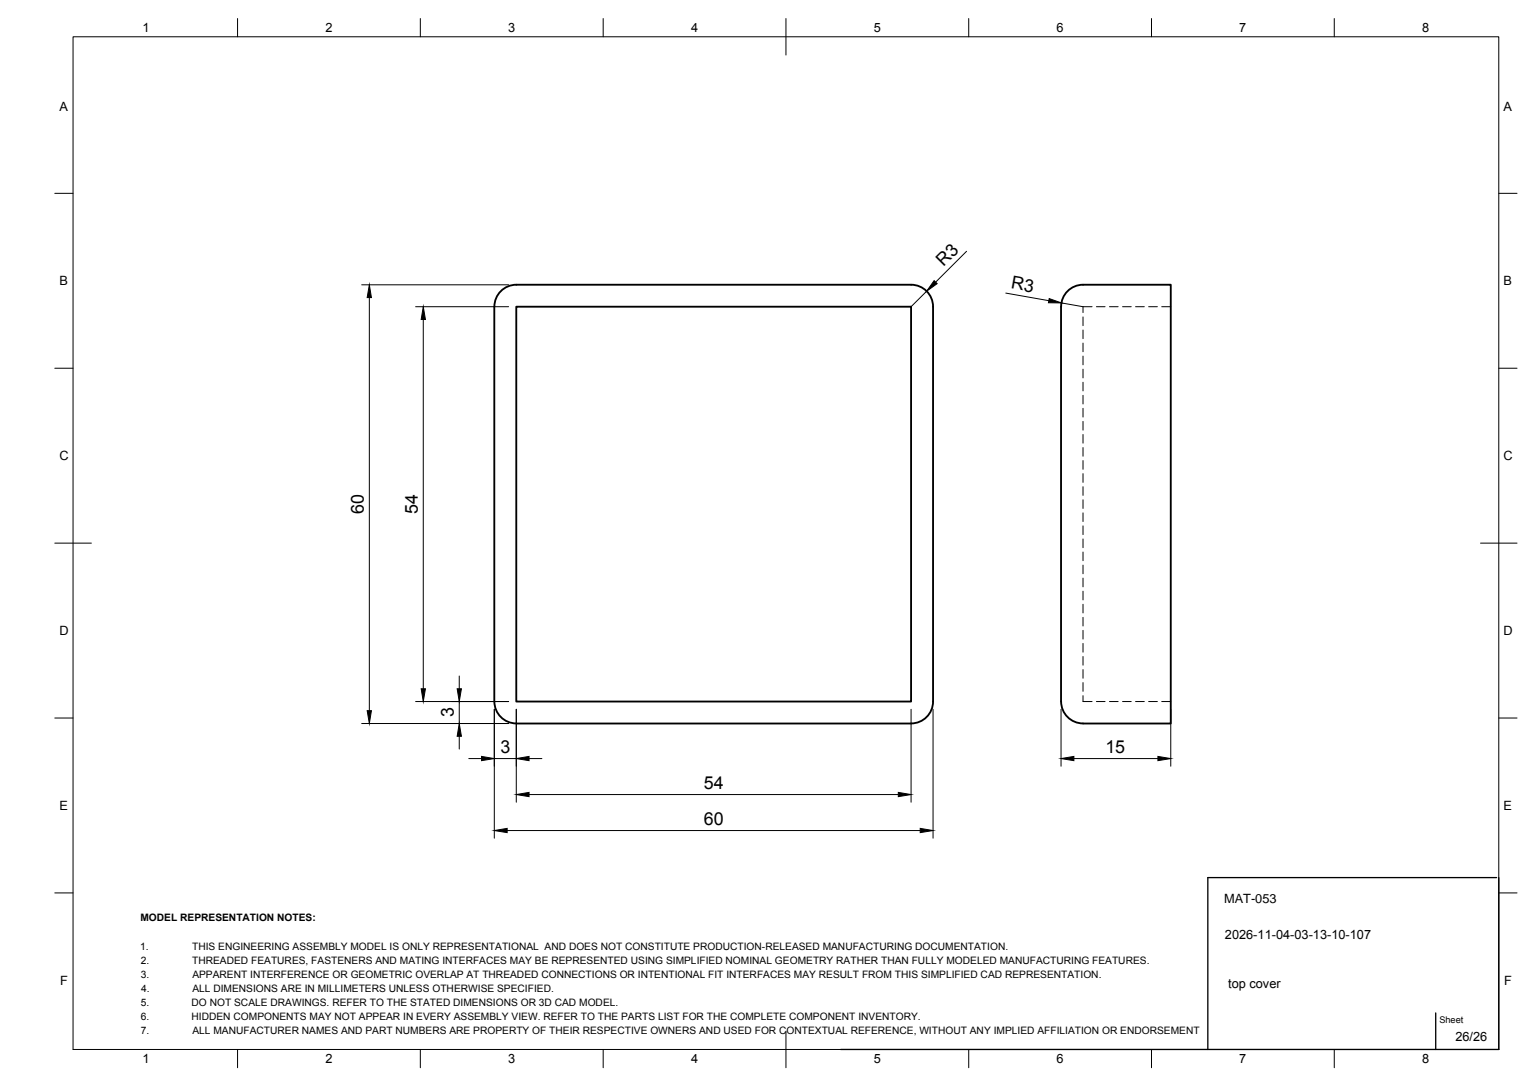
ISO-10303-21;
HEADER;
FILE_DESCRIPTION (('STEP AP214'),
    '1' );
FILE_NAME ('top cover.step',
    '2026-10-10T03:43:58',
    ( '' ),
    ( '' ),
    'SwSTEP 2.0',
    'SolidWorks 2026',
    '' );
FILE_SCHEMA (( 'AUTOMOTIVE_DESIGN' ));
ENDSEC;

DATA;
#205=DIRECTION ( 'NONE',  ( 0.000000000000000000, 0.000000000000000000, -1.000000000000000000 ) ) ;
#232=CARTESIAN_POINT ( 'NONE',  ( -30.00000000000000355, 26.99999999999999289, 12.00000000000000000 ) ) ;
#298=DIRECTION ( 'NONE',  ( 0.000000000000000000, 1.000000000000000000, 0.000000000000000000 ) ) ;
#580=CARTESIAN_POINT ( 'NONE',  ( 0.000000000000000000, 0.000000000000000000, 0.000000000000000000 ) ) ;
#658=DIRECTION ( 'NONE',  ( 0.000000000000000000, 1.000000000000000000, 0.000000000000000000 ) ) ;
#710=ORIENTED_EDGE ( 'NONE', *, *, #12281, .T. ) ;
#818=VECTOR ( 'NONE', #14052, 1000.000000000000000 ) ;
#1029=CARTESIAN_POINT ( 'NONE',  ( 26.99999999999999645, -27.00000000000000355, 12.00000000000000000 ) ) ;
#1414=ORIENTED_EDGE ( 'NONE', *, *, #50736, .T. ) ;
#1463=DIRECTION ( 'NONE',  ( 0.000000000000000000, -1.000000000000000000, 0.000000000000000000 ) ) ;
#1569=CARTESIAN_POINT ( 'NONE',  ( 26.99999999999999645, 0.000000000000000000, 15.00000000000000000 ) ) ;
#1686=CIRCLE ( 'NONE', #47705, 2.999999999999999112 ) ;
#1835=CARTESIAN_POINT ( 'NONE',  ( -27.00000000000000355, -27.00000000000000355, 15.00000000000000000 ) ) ;
#1860=LINE ( 'NONE', #18024, #9010 ) ;
#1950=ORIENTED_EDGE ( 'NONE', *, *, #16118, .F. ) ;
#2102=ORIENTED_EDGE ( 'NONE', *, *, #62336, .T. ) ;
#2271=FACE_OUTER_BOUND ( 'NONE', #44764, .T. ) ;
#2303=EDGE_CURVE ( 'NONE', #6058, #28877, #22222, .T. ) ;
#2927=ORIENTED_EDGE ( 'NONE', *, *, #30408, .T. ) ;
#3081=AXIS2_PLACEMENT_3D ( 'NONE', #1029, #66114, #17904 ) ;
#3101=EDGE_LOOP ( 'NONE', ( #24985, #13574, #25623 ) ) ;
#3252=DIRECTION ( 'NONE',  ( 0.000000000000000000, -1.000000000000000000, 0.000000000000000000 ) ) ;
#3314=EDGE_CURVE ( 'NONE', #69327, #44889, #32443, .T. ) ;
#3324=DIRECTION ( 'NONE',  ( -0.000000000000000000, -0.000000000000000000, -1.000000000000000000 ) ) ;
#3439=ADVANCED_FACE ( 'NONE', ( #7097 ), #12728, .T. ) ;
#3520=CARTESIAN_POINT ( 'NONE',  ( 26.99999999999999645, 0.000000000000000000, -0.000000000000000000 ) ) ;
#3667=CARTESIAN_POINT ( 'NONE',  ( -27.00000000000000355, 26.99999999999999645, 0.000000000000000000 ) ) ;
#3801=DIRECTION ( 'NONE',  ( -1.000000000000000000, -1.156482317317871725E-15, 0.000000000000000000 ) ) ;
#3891=ORIENTED_EDGE ( 'NONE', *, *, #46841, .F. ) ;
#4008=ORIENTED_EDGE ( 'NONE', *, *, #30408, .F. ) ;
#4241=EDGE_CURVE ( 'NONE', #32499, #62713, #15839, .T. ) ;
#4403=ORIENTED_EDGE ( 'NONE', *, *, #17309, .T. ) ;
#4446=DIRECTION ( 'NONE',  ( 0.000000000000000000, 0.000000000000000000, -1.000000000000000000 ) ) ;
#4489=LINE ( 'NONE', #19627, #58799 ) ;
#4810=DIRECTION ( 'NONE',  ( 0.000000000000000000, 0.000000000000000000, 1.000000000000000000 ) ) ;
#4904=EDGE_CURVE ( 'NONE', #26503, #8633, #55459, .T. ) ;
#5040=CARTESIAN_POINT ( 'NONE',  ( 29.99999999999999645, -27.00000000000000355, 15.00000000000000000 ) ) ;
#5156=ORIENTED_EDGE ( 'NONE', *, *, #23205, .T. ) ;
#5210=PLANE ( 'NONE',  #52619 ) ;
#5318=DIRECTION ( 'NONE',  ( 0.000000000000000000, 0.000000000000000000, -1.000000000000000000 ) ) ;
#5366=AXIS2_PLACEMENT_3D ( 'NONE', #65979, #17774, #7580 ) ;
#5409=ORIENTED_EDGE ( 'NONE', *, *, #63357, .T. ) ;
#5648=CARTESIAN_POINT ( 'NONE',  ( -27.00000000000000355, 26.99999999999999289, 0.000000000000000000 ) ) ;
#5733=VECTOR ( 'NONE', #47729, 1000.000000000000000 ) ;
#5803=ORIENTED_EDGE ( 'NONE', *, *, #46794, .F. ) ;
#5843=DIRECTION ( 'NONE',  ( -1.000000000000000000, 0.000000000000000000, -0.000000000000000000 ) ) ;
#5940=CARTESIAN_POINT ( 'NONE',  ( 26.99999999999999289, -30.00000000000000355, 0.000000000000000000 ) ) ;
#5961=DIRECTION ( 'NONE',  ( 0.000000000000000000, 0.000000000000000000, -1.000000000000000000 ) ) ;
#6058=VERTEX_POINT ( 'NONE', #3667 ) ;
#6102=ORIENTED_EDGE ( 'NONE', *, *, #58756, .F. ) ;
#6143=DIRECTION ( 'NONE',  ( 0.000000000000000000, 0.000000000000000000, -1.000000000000000000 ) ) ;
#6198=FACE_OUTER_BOUND ( 'NONE', #21474, .T. ) ;
#6225=VERTEX_POINT ( 'NONE', #41647 ) ;
#6428=VECTOR ( 'NONE', #48833, 1000.000000000000000 ) ;
#6478=ORIENTED_EDGE ( 'NONE', *, *, #62336, .F. ) ;
#6480=ORIENTED_EDGE ( 'NONE', *, *, #50724, .F. ) ;
#6516=EDGE_CURVE ( 'NONE', #6225, #40175, #1686, .T. ) ;
#6716=FACE_OUTER_BOUND ( 'NONE', #43158, .T. ) ;
#6823=CARTESIAN_POINT ( 'NONE',  ( 0.000000000000000000, -27.00000000000000355, 15.00000000000000000 ) ) ;
#6825=DIRECTION ( 'NONE',  ( -0.000000000000000000, -0.000000000000000000, 1.000000000000000000 ) ) ;
#6889=ORIENTED_EDGE ( 'NONE', *, *, #66647, .F. ) ;
#7011=DIRECTION ( 'NONE',  ( 1.000000000000000000, 0.000000000000000000, 0.000000000000000000 ) ) ;
#7097=FACE_OUTER_BOUND ( 'NONE', #42212, .T. ) ;
#7102=VECTOR ( 'NONE', #45225, 1000.000000000000000 ) ;
#7438=ORIENTED_EDGE ( 'NONE', *, *, #22139, .T. ) ;
#7471=CIRCLE ( 'NONE', #49967, 2.999999999999999112 ) ;
#7580=DIRECTION ( 'NONE',  ( 0.000000000000000000, -0.000000000000000000, -1.000000000000000000 ) ) ;
#7623=AXIS2_PLACEMENT_3D ( 'NONE', #12347, #50333, #60872 ) ;
#7667=VERTEX_POINT ( 'NONE', #19524 ) ;
#7674=CARTESIAN_POINT ( 'NONE',  ( 26.99999999999999289, 26.99999999999999645, 12.00000000000000000 ) ) ;
#8001=LINE ( 'NONE', #29456, #37178 ) ;
#8141=CARTESIAN_POINT ( 'NONE',  ( -27.00000000000000355, -30.00000000000000355, 15.00000000000000000 ) ) ;
#8234=CYLINDRICAL_SURFACE ( 'NONE', #53074, 2.999999999999999112 ) ;
#8319=DIRECTION ( 'NONE',  ( 1.000000000000000000, 0.000000000000000000, 0.000000000000000000 ) ) ;
#8334=FACE_OUTER_BOUND ( 'NONE', #46485, .T. ) ;
#8423=ADVANCED_FACE ( 'NONE', ( #66101 ), #17538, .F. ) ;
#8496=LINE ( 'NONE', #45780, #36770 ) ;
#8633=VERTEX_POINT ( 'NONE', #11470 ) ;
#8718=AXIS2_PLACEMENT_3D ( 'NONE', #29906, #55232, #39077 ) ;
#8728=FACE_OUTER_BOUND ( 'NONE', #54277, .T. ) ;
#8810=ORIENTED_EDGE ( 'NONE', *, *, #54510, .T. ) ;
#8945=ORIENTED_EDGE ( 'NONE', *, *, #65993, .T. ) ;
#9010=VECTOR ( 'NONE', #54598, 1000.000000000000000 ) ;
#9074=PRODUCT_DEFINITION_SHAPE ( 'NONE', 'NONE',  #55565 ) ;
#9081=VERTEX_POINT ( 'NONE', #5940 ) ;
#9480=EDGE_CURVE ( 'NONE', #41324, #25791, #48125, .T. ) ;
#9811=CIRCLE ( 'NONE', #12060, 2.999999999999999112 ) ;
#9857=ADVANCED_FACE ( 'NONE', ( #21322 ), #65637, .T. ) ;
#9955=PRODUCT_DEFINITION_CONTEXT ( 'detailed design', #26937, 'design' ) ;
#10261=CARTESIAN_POINT ( 'NONE',  ( 26.99999999999999645, 26.99999999999999645, 12.00000000000000000 ) ) ;
#10445=CARTESIAN_POINT ( 'NONE',  ( 26.99999999999999645, 26.99999999999999645, 12.00000000000000000 ) ) ;
#10700=ADVANCED_FACE ( 'NONE', ( #6716 ), #19613, .T. ) ;
#10784=ADVANCED_FACE ( 'NONE', ( #8728 ), #33803, .T. ) ;
#10889=CIRCLE ( 'NONE', #3081, 2.999999999999999112 ) ;
#11030=CARTESIAN_POINT ( 'NONE',  ( 26.99999999999999645, -30.00000000000000355, 15.00000000000000000 ) ) ;
#11039=ORIENTED_EDGE ( 'NONE', *, *, #23029, .T. ) ;
#11086=ORIENTED_EDGE ( 'NONE', *, *, #66647, .T. ) ;
#11217=LINE ( 'NONE', #32684, #6428 ) ;
#11234=VECTOR ( 'NONE', #23749, 1000.000000000000000 ) ;
#11470=CARTESIAN_POINT ( 'NONE',  ( -30.00000000000000355, -27.00000000000000355, 0.000000000000000000 ) ) ;
#11537=PLANE ( 'NONE',  #37652 ) ;
#12060=AXIS2_PLACEMENT_3D ( 'NONE', #26984, #27675, #49116 ) ;
#12281=EDGE_CURVE ( 'NONE', #9081, #43408, #15395, .T. ) ;
#12347=CARTESIAN_POINT ( 'NONE',  ( -30.00000000000000355, 26.99999999999999645, 15.00000000000000000 ) ) ;
#12478=LINE ( 'NONE', #1569, #18550 ) ;
#12484=CARTESIAN_POINT ( 'NONE',  ( -30.00000000000000355, -27.00000000000000355, 12.00000000000000000 ) ) ;
#12728=CYLINDRICAL_SURFACE ( 'NONE', #65623, 2.999999999999999112 ) ;
#12815=UNCERTAINTY_MEASURE_WITH_UNIT (LENGTH_MEASURE( 1.000000000000000082E-05 ), #48462, 'distance_accuracy_value', 'NONE');
#12853=DIRECTION ( 'NONE',  ( -0.000000000000000000, -0.000000000000000000, 1.000000000000000000 ) ) ;
#12906=ADVANCED_FACE ( 'NONE', ( #19001 ), #17611, .T. ) ;
#12964=ADVANCED_FACE ( 'NONE', ( #41498 ), #31295, .T. ) ;
#13056=CARTESIAN_POINT ( 'NONE',  ( 29.99999999999999645, -30.00000000000000355, 15.00000000000000000 ) ) ;
#13156=EDGE_LOOP ( 'NONE', ( #33249, #52496, #29073, #69310 ) ) ;
#13179=VECTOR ( 'NONE', #67585, 1000.000000000000000 ) ;
#13198=CARTESIAN_POINT ( 'NONE',  ( 29.99999999999999645, 26.99999999999999289, 15.00000000000000000 ) ) ;
#13396=FACE_OUTER_BOUND ( 'NONE', #32596, .T. ) ;
#13574=ORIENTED_EDGE ( 'NONE', *, *, #33002, .T. ) ;
#13635=ADVANCED_FACE ( 'NONE', ( #13396 ), #62265, .T. ) ;
#13692=VECTOR ( 'NONE', #25426, 1000.000000000000000 ) ;
#13696=ORIENTED_EDGE ( 'NONE', *, *, #42477, .T. ) ;
#13708=ORIENTED_EDGE ( 'NONE', *, *, #25060, .F. ) ;
#13830=AXIS2_PLACEMENT_3D ( 'NONE', #48385, #55427, #44883 ) ;
#13919=CIRCLE ( 'NONE', #29629, 2.999999999999999112 ) ;
#14052=DIRECTION ( 'NONE',  ( 1.000000000000000000, 0.000000000000000000, 0.000000000000000000 ) ) ;
#14415=ORIENTED_EDGE ( 'NONE', *, *, #50724, .T. ) ;
#14417=LINE ( 'NONE', #29901, #51494 ) ;
#14459=DIRECTION ( 'NONE',  ( 0.000000000000000000, 0.000000000000000000, -1.000000000000000000 ) ) ;
#14478=CIRCLE ( 'NONE', #21293, 2.999999999999999112 ) ;
#14630=ORIENTED_EDGE ( 'NONE', *, *, #6516, .F. ) ;
#14733=VECTOR ( 'NONE', #50808, 1000.000000000000000 ) ;
#14750=DIRECTION ( 'NONE',  ( 0.000000000000000000, 0.000000000000000000, 1.000000000000000000 ) ) ;
#14758=DIRECTION ( 'NONE',  ( -1.000000000000000000, 0.000000000000000000, 0.000000000000000000 ) ) ;
#14846=CARTESIAN_POINT ( 'NONE',  ( 0.000000000000000000, 26.99999999999999645, 0.000000000000000000 ) ) ;
#14880=CARTESIAN_POINT ( 'NONE',  ( -30.00000000000000355, -30.00000000000000355, 12.00000000000000000 ) ) ;
#14925=AXIS2_PLACEMENT_3D ( 'NONE', #580, #32930, #5843 ) ;
#15172=CIRCLE ( 'NONE', #65745, 2.999999999999999112 ) ;
#15255=EDGE_LOOP ( 'NONE', ( #31860, #60299, #4403, #51256 ) ) ;
#15269=EDGE_LOOP ( 'NONE', ( #5409, #23940, #8810, #19099 ) ) ;
#15349=CARTESIAN_POINT ( 'NONE',  ( 26.99999999999999289, 26.99999999999999645, 0.000000000000000000 ) ) ;
#15395=LINE ( 'NONE', #44096, #62596 ) ;
#15581=VECTOR ( 'NONE', #57340, 1000.000000000000000 ) ;
#15839=LINE ( 'NONE', #64363, #26189 ) ;
#16028=( GEOMETRIC_REPRESENTATION_CONTEXT ( 3 ) GLOBAL_UNCERTAINTY_ASSIGNED_CONTEXT ( ( #12815 ) ) GLOBAL_UNIT_ASSIGNED_CONTEXT ( ( #48462, #43201, #37241 ) ) REPRESENTATION_CONTEXT ( 'NONE', 'WORKASPACE' ) );
#16037=DIRECTION ( 'NONE',  ( -0.000000000000000000, -1.000000000000000000, -0.000000000000000000 ) ) ;
#16118=EDGE_CURVE ( 'NONE', #6225, #52460, #57437, .T. ) ;
#16138=FILL_AREA_STYLE ('',( #37940 ) ) ;
#16158=EDGE_LOOP ( 'NONE', ( #47934, #54871, #19275, #17353 ) ) ;
#16540=DIRECTION ( 'NONE',  ( 0.000000000000000000, 0.000000000000000000, 1.000000000000000000 ) ) ;
#16832=DIRECTION ( 'NONE',  ( -1.000000000000000000, 0.000000000000000000, -0.000000000000000000 ) ) ;
#16893=CARTESIAN_POINT ( 'NONE',  ( 26.99999999999999645, -27.00000000000000355, 15.00000000000000000 ) ) ;
#17309=EDGE_CURVE ( 'NONE', #39573, #51452, #60293, .T. ) ;
#17353=ORIENTED_EDGE ( 'NONE', *, *, #38024, .F. ) ;
#17522=AXIS2_PLACEMENT_3D ( 'NONE', #10445, #68838, #3801 ) ;
#17538=PLANE ( 'NONE',  #29861 ) ;
#17561=CARTESIAN_POINT ( 'NONE',  ( -27.00000000000000355, -27.00000000000000355, 12.00000000000000000 ) ) ;
#17611=PLANE ( 'NONE',  #8718 ) ;
#17774=DIRECTION ( 'NONE',  ( 0.000000000000000000, -1.000000000000000000, 0.000000000000000000 ) ) ;
#17904=DIRECTION ( 'NONE',  ( 0.000000000000000000, 0.000000000000000000, -1.000000000000000000 ) ) ;
#18024=CARTESIAN_POINT ( 'NONE',  ( -27.00000000000000355, -30.00000000000000355, 12.00000000000000000 ) ) ;
#18121=FACE_OUTER_BOUND ( 'NONE', #15269, .T. ) ;
#18189=CARTESIAN_POINT ( 'NONE',  ( -27.00000000000000355, 0.000000000000000000, 12.00000000000000000 ) ) ;
#18295=DIRECTION ( 'NONE',  ( 0.000000000000000000, 0.000000000000000000, -1.000000000000000000 ) ) ;
#18314=DIRECTION ( 'NONE',  ( 0.000000000000000000, 0.000000000000000000, 1.000000000000000000 ) ) ;
#18380=CARTESIAN_POINT ( 'NONE',  ( -27.00000000000000355, 0.000000000000000000, 15.00000000000000000 ) ) ;
#18492=AXIS2_PLACEMENT_3D ( 'NONE', #7674, #66771, #66427 ) ;
#18550=VECTOR ( 'NONE', #66655, 1000.000000000000000 ) ;
#18804=EDGE_CURVE ( 'NONE', #8633, #64962, #45182, .T. ) ;
#19001=FACE_OUTER_BOUND ( 'NONE', #64825, .T. ) ;
#19099=ORIENTED_EDGE ( 'NONE', *, *, #46794, .T. ) ;
#19215=CYLINDRICAL_SURFACE ( 'NONE', #39889, 2.999999999999999112 ) ;
#19275=ORIENTED_EDGE ( 'NONE', *, *, #65275, .F. ) ;
#19323=VERTEX_POINT ( 'NONE', #40685 ) ;
#19413=ORIENTED_EDGE ( 'NONE', *, *, #22139, .F. ) ;
#19469=CARTESIAN_POINT ( 'NONE',  ( 26.99999999999999645, 0.000000000000000000, 12.00000000000000000 ) ) ;
#19485=CARTESIAN_POINT ( 'NONE',  ( -30.00000000000000355, -27.00000000000000355, 15.00000000000000000 ) ) ;
#19524=CARTESIAN_POINT ( 'NONE',  ( -27.00000000000000355, -30.00000000000000355, 12.00000000000000000 ) ) ;
#19613=SPHERICAL_SURFACE ( 'NONE', #23333, 3.000000000000000000 ) ;
#19627=CARTESIAN_POINT ( 'NONE',  ( -30.00000000000000355, 26.99999999999999645, 12.00000000000000000 ) ) ;
#19872=EDGE_CURVE ( 'NONE', #6225, #39573, #57397, .T. ) ;
#19906=VECTOR ( 'NONE', #12853, 1000.000000000000000 ) ;
#20346=CARTESIAN_POINT ( 'NONE',  ( -27.00000000000000355, -30.00000000000000355, 15.00000000000000000 ) ) ;
#20503=LINE ( 'NONE', #14880, #48624 ) ;
#20784=ADVANCED_FACE ( 'NONE', ( #63984 ), #43899, .T. ) ;
#20791=MANIFOLD_SOLID_BREP ( 'Shell1', #42893 ) ;
#20967=DIRECTION ( 'NONE',  ( -1.000000000000000000, 0.000000000000000000, 0.000000000000000000 ) ) ;
#21082=ORIENTED_EDGE ( 'NONE', *, *, #30023, .T. ) ;
#21293=AXIS2_PLACEMENT_3D ( 'NONE', #39648, #54767, #34030 ) ;
#21294=DIRECTION ( 'NONE',  ( -1.000000000000000000, 0.000000000000000000, 0.000000000000000000 ) ) ;
#21320=DIRECTION ( 'NONE',  ( -1.000000000000000000, -0.000000000000000000, -0.000000000000000000 ) ) ;
#21321=ADVANCED_FACE ( 'NONE', ( #59647, #38206 ), #42447, .T. ) ;
#21322=FACE_OUTER_BOUND ( 'NONE', #56192, .T. ) ;
#21333=FACE_OUTER_BOUND ( 'NONE', #52946, .T. ) ;
#21352=ADVANCED_FACE ( 'NONE', ( #6198 ), #43473, .T. ) ;
#21422=ADVANCED_FACE ( 'NONE', ( #21333 ), #26957, .T. ) ;
#21428=EDGE_CURVE ( 'NONE', #64962, #40175, #32250, .T. ) ;
#21474=EDGE_LOOP ( 'NONE', ( #13696, #62459, #1950, #30513 ) ) ;
#21793=CARTESIAN_POINT ( 'NONE',  ( -27.00000000000000355, 29.99999999999999645, 0.000000000000000000 ) ) ;
#22018=CARTESIAN_POINT ( 'NONE',  ( 26.99999999999999645, -27.00000000000000355, 15.00000000000000000 ) ) ;
#22139=EDGE_CURVE ( 'NONE', #55869, #25791, #4489, .T. ) ;
#22181=ORIENTED_EDGE ( 'NONE', *, *, #55920, .F. ) ;
#22222=LINE ( 'NONE', #28185, #62196 ) ;
#22231=DIRECTION ( 'NONE',  ( 0.000000000000000000, 0.000000000000000000, -1.000000000000000000 ) ) ;
#22375=DIRECTION ( 'NONE',  ( 0.000000000000000000, 0.000000000000000000, 1.000000000000000000 ) ) ;
#22511=CARTESIAN_POINT ( 'NONE',  ( -27.00000000000000355, -27.00000000000000355, 15.00000000000000000 ) ) ;
#22720=CARTESIAN_POINT ( 'NONE',  ( -27.00000000000000355, -27.00000000000000355, 12.00000000000000000 ) ) ;
#23029=EDGE_CURVE ( 'NONE', #7667, #26503, #45423, .T. ) ;
#23205=EDGE_CURVE ( 'NONE', #28877, #59754, #42563, .T. ) ;
#23333=AXIS2_PLACEMENT_3D ( 'NONE', #28881, #28161, #66185 ) ;
#23743=CARTESIAN_POINT ( 'NONE',  ( 29.99999999999999645, -27.00000000000000355, 0.000000000000000000 ) ) ;
#23749=DIRECTION ( 'NONE',  ( 0.000000000000000000, 0.000000000000000000, -1.000000000000000000 ) ) ;
#23940=ORIENTED_EDGE ( 'NONE', *, *, #55920, .T. ) ;
#24075=CIRCLE ( 'NONE', #18492, 2.999999999999999112 ) ;
#24302=PLANE ( 'NONE',  #33156 ) ;
#24695=ADVANCED_FACE ( 'NONE', ( #8334 ), #19215, .T. ) ;
#24734=DIRECTION ( 'NONE',  ( 0.000000000000000000, -0.000000000000000000, 1.000000000000000000 ) ) ;
#24976=EDGE_CURVE ( 'NONE', #43408, #44889, #29799, .T. ) ;
#24985=ORIENTED_EDGE ( 'NONE', *, *, #58756, .T. ) ;
#24993=STYLED_ITEM ( 'NONE', ( #58355 ), #20791 ) ;
#25060=EDGE_CURVE ( 'NONE', #51452, #42318, #12478, .T. ) ;
#25151=AXIS2_PLACEMENT_3D ( 'NONE', #31684, #69315, #60843 ) ;
#25426=DIRECTION ( 'NONE',  ( -1.000000000000000000, 0.000000000000000000, 0.000000000000000000 ) ) ;
#25582=DIRECTION ( 'NONE',  ( 0.000000000000000000, 1.000000000000000000, 0.000000000000000000 ) ) ;
#25623=ORIENTED_EDGE ( 'NONE', *, *, #50443, .F. ) ;
#25689=LINE ( 'NONE', #3520, #15581 ) ;
#25714=DIRECTION ( 'NONE',  ( 1.000000000000000000, -0.000000000000000000, 0.000000000000000000 ) ) ;
#25791=VERTEX_POINT ( 'NONE', #26067 ) ;
#25812=AXIS2_PLACEMENT_3D ( 'NONE', #28884, #50672, #29224 ) ;
#25890=PRODUCT_CONTEXT ( 'NONE', #58769, 'mechanical' ) ;
#25918=LINE ( 'NONE', #53306, #62997 ) ;
#26000=CARTESIAN_POINT ( 'NONE',  ( -27.00000000000000355, 26.99999999999999289, 12.00000000000000000 ) ) ;
#26067=CARTESIAN_POINT ( 'NONE',  ( 26.99999999999999645, 26.99999999999999645, 12.00000000000000000 ) ) ;
#26189=VECTOR ( 'NONE', #63343, 1000.000000000000000 ) ;
#26232=CYLINDRICAL_SURFACE ( 'NONE', #50132, 2.999999999999999112 ) ;
#26328=DIRECTION ( 'NONE',  ( 0.000000000000000000, 0.000000000000000000, -1.000000000000000000 ) ) ;
#26357=CARTESIAN_POINT ( 'NONE',  ( 26.99999999999999289, 29.99999999999999645, 0.000000000000000000 ) ) ;
#26389=ORIENTED_EDGE ( 'NONE', *, *, #43751, .T. ) ;
#26423=ORIENTED_EDGE ( 'NONE', *, *, #50443, .T. ) ;
#26503=VERTEX_POINT ( 'NONE', #35598 ) ;
#26528=DIRECTION ( 'NONE',  ( -1.000000000000000000, 0.000000000000000000, 0.000000000000000000 ) ) ;
#26668=DIRECTION ( 'NONE',  ( 1.000000000000000000, 0.000000000000000000, 0.000000000000000000 ) ) ;
#26860=AXIS2_PLACEMENT_3D ( 'NONE', #49201, #37972, #7011 ) ;
#26910=ADVANCED_FACE ( 'NONE', ( #61229 ), #24302, .F. ) ;
#26937=APPLICATION_CONTEXT ( 'automotive_design' ) ;
#26957=SPHERICAL_SURFACE ( 'NONE', #13830, 3.000000000000000000 ) ;
#26984=CARTESIAN_POINT ( 'NONE',  ( -27.00000000000000355, 26.99999999999999645, 12.00000000000000000 ) ) ;
#27010=ADVANCED_FACE ( 'NONE', ( #48816 ), #11537, .F. ) ;
#27026=AXIS2_PLACEMENT_3D ( 'NONE', #41140, #56624, #18295 ) ;
#27068=ORIENTED_EDGE ( 'NONE', *, *, #30420, .T. ) ;
#27182=VECTOR ( 'NONE', #54516, 1000.000000000000000 ) ;
#27248=CARTESIAN_POINT ( 'NONE',  ( -30.00000000000000355, 29.99999999999999645, 12.00000000000000000 ) ) ;
#27377=SURFACE_STYLE_FILL_AREA ( #16138 ) ;
#27456=EDGE_LOOP ( 'NONE', ( #49518, #62100, #56589, #22181 ) ) ;
#27675=DIRECTION ( 'NONE',  ( 0.000000000000000000, -0.000000000000000000, 1.000000000000000000 ) ) ;
#27696=EDGE_LOOP ( 'NONE', ( #2927, #11086, #60441, #28815 ) ) ;
#27909=PLANE ( 'NONE',  #47841 ) ;
#27999=CARTESIAN_POINT ( 'NONE',  ( -30.00000000000000355, -30.00000000000000355, 12.00000000000000000 ) ) ;
#28096=CARTESIAN_POINT ( 'NONE',  ( 26.99999999999999289, 29.99999999999999645, 15.00000000000000000 ) ) ;
#28161=DIRECTION ( 'NONE',  ( 1.000000000000000000, 0.000000000000000000, 0.000000000000000000 ) ) ;
#28185=CARTESIAN_POINT ( 'NONE',  ( -27.00000000000000355, 0.000000000000000000, -0.000000000000000000 ) ) ;
#28196=DIRECTION ( 'NONE',  ( -1.000000000000000000, 0.000000000000000000, 0.000000000000000000 ) ) ;
#28288=SHAPE_REPRESENTATION_RELATIONSHIP ( 'NONE' , 'NONE' ,  #31639, #32386 ) ;
#28319=ADVANCED_FACE ( 'NONE', ( #41781 ), #62893, .T. ) ;
#28482=EDGE_LOOP ( 'NONE', ( #6478, #66068, #6480, #57491, #36541, #8945, #38878, #60954 ) ) ;
#28660=CARTESIAN_POINT ( 'NONE',  ( 26.99999999999999645, -27.00000000000000355, 12.00000000000000000 ) ) ;
#28671=CARTESIAN_POINT ( 'NONE',  ( 26.99999999999999289, 29.99999999999999645, 12.00000000000000000 ) ) ;
#28815=ORIENTED_EDGE ( 'NONE', *, *, #38024, .T. ) ;
#28877=VERTEX_POINT ( 'NONE', #56670 ) ;
#28881=CARTESIAN_POINT ( 'NONE',  ( -27.00000000000000355, 26.99999999999999645, 12.00000000000000000 ) ) ;
#28884=CARTESIAN_POINT ( 'NONE',  ( 0.000000000000000000, -27.00000000000000355, 12.00000000000000000 ) ) ;
#29073=ORIENTED_EDGE ( 'NONE', *, *, #3314, .T. ) ;
#29224=DIRECTION ( 'NONE',  ( 0.000000000000000000, 0.000000000000000000, -1.000000000000000000 ) ) ;
#29456=CARTESIAN_POINT ( 'NONE',  ( -30.00000000000000355, -30.00000000000000355, 0.000000000000000000 ) ) ;
#29629=AXIS2_PLACEMENT_3D ( 'NONE', #54138, #5961, #48857 ) ;
#29640=VECTOR ( 'NONE', #14459, 1000.000000000000000 ) ;
#29677=ORIENTED_EDGE ( 'NONE', *, *, #21428, .F. ) ;
#29777=DIRECTION ( 'NONE',  ( 0.000000000000000000, 0.000000000000000000, -1.000000000000000000 ) ) ;
#29799=CIRCLE ( 'NONE', #64643, 2.999999999999999112 ) ;
#29803=( GEOMETRIC_REPRESENTATION_CONTEXT ( 3 ) GLOBAL_UNCERTAINTY_ASSIGNED_CONTEXT ( ( #35303 ) ) GLOBAL_UNIT_ASSIGNED_CONTEXT ( ( #55012, #39545, #50099 ) ) REPRESENTATION_CONTEXT ( 'NONE', 'WORKASPACE' ) );
#29861=AXIS2_PLACEMENT_3D ( 'NONE', #49892, #55165, #16832 ) ;
#29901=CARTESIAN_POINT ( 'NONE',  ( -30.00000000000000355, 29.99999999999999645, 0.000000000000000000 ) ) ;
#29906=CARTESIAN_POINT ( 'NONE',  ( 0.000000000000000000, 0.000000000000000000, 12.00000000000000000 ) ) ;
#29954=VECTOR ( 'NONE', #14750, 1000.000000000000000 ) ;
#30023=EDGE_CURVE ( 'NONE', #52460, #40175, #9811, .T. ) ;
#30400=CARTESIAN_POINT ( 'NONE',  ( -27.00000000000000355, -27.00000000000000355, 12.00000000000000000 ) ) ;
#30408=EDGE_CURVE ( 'NONE', #19323, #58514, #41537, .T. ) ;
#30420=EDGE_CURVE ( 'NONE', #40175, #48508, #8496, .T. ) ;
#30513=ORIENTED_EDGE ( 'NONE', *, *, #46788, .F. ) ;
#30582=CARTESIAN_POINT ( 'NONE',  ( -30.00000000000000355, -30.00000000000000355, 0.000000000000000000 ) ) ;
#30781=CARTESIAN_POINT ( 'NONE',  ( 26.99999999999999645, -30.00000000000000355, 12.00000000000000000 ) ) ;
#31081=DIRECTION ( 'NONE',  ( -1.000000000000000000, 0.000000000000000000, -0.000000000000000000 ) ) ;
#31295=CYLINDRICAL_SURFACE ( 'NONE', #65063, 2.999999999999999112 ) ;
#31331=CARTESIAN_POINT ( 'NONE',  ( 0.000000000000000000, -27.00000000000000355, -0.000000000000000000 ) ) ;
#31628=CARTESIAN_POINT ( 'NONE',  ( 26.99999999999999645, -27.00000000000000355, 12.00000000000000000 ) ) ;
#31631=DIRECTION ( 'NONE',  ( 0.000000000000000000, -0.000000000000000000, 1.000000000000000000 ) ) ;
#31639=SHAPE_REPRESENTATION ( 'top cover', ( #66832 ), #29803 ) ;
#31684=CARTESIAN_POINT ( 'NONE',  ( -27.00000000000000355, -27.00000000000000355, 0.000000000000000000 ) ) ;
#31705=DIRECTION ( 'NONE',  ( -1.000000000000000000, 0.000000000000000000, 0.000000000000000000 ) ) ;
#31860=ORIENTED_EDGE ( 'NONE', *, *, #46788, .T. ) ;
#31914=ADVANCED_FACE ( 'NONE', ( #47081 ), #5210, .T. ) ;
#31962=DIRECTION ( 'NONE',  ( -0.000000000000000000, -1.000000000000000000, 1.156482317317871725E-15 ) ) ;
#32096=DIRECTION ( 'NONE',  ( -0.000000000000000000, -1.000000000000000000, -0.000000000000000000 ) ) ;
#32152=PRODUCT_DEFINITION_FORMATION_WITH_SPECIFIED_SOURCE ( 'ANY', '', #37747, .NOT_KNOWN. ) ;
#32203=CARTESIAN_POINT ( 'NONE',  ( -27.00000000000000355, 26.99999999999999289, 15.00000000000000000 ) ) ;
#32250=LINE ( 'NONE', #27999, #7102 ) ;
#32375=VERTEX_POINT ( 'NONE', #28671 ) ;
#32386=ADVANCED_BREP_SHAPE_REPRESENTATION ( '', ( #20791, #66832 ), #29803 ) ;
#32443=LINE ( 'NONE', #53871, #40909 ) ;
#32499=VERTEX_POINT ( 'NONE', #23743 ) ;
#32596=EDGE_LOOP ( 'NONE', ( #67958, #61971, #6102, #68427 ) ) ;
#32658=EDGE_CURVE ( 'NONE', #44889, #32499, #58842, .T. ) ;
#32684=CARTESIAN_POINT ( 'NONE',  ( 0.000000000000000000, 26.99999999999999645, 15.00000000000000000 ) ) ;
#32930=DIRECTION ( 'NONE',  ( 0.000000000000000000, 0.000000000000000000, -1.000000000000000000 ) ) ;
#32965=ADVANCED_FACE ( 'NONE', ( #55660 ), #39830, .T. ) ;
#33002=EDGE_CURVE ( 'NONE', #39573, #64962, #38099, .T. ) ;
#33156=AXIS2_PLACEMENT_3D ( 'NONE', #13056, #66522, #18314 ) ;
#33220=ORIENTED_EDGE ( 'NONE', *, *, #52083, .F. ) ;
#33249=ORIENTED_EDGE ( 'NONE', *, *, #4241, .T. ) ;
#33528=CARTESIAN_POINT ( 'NONE',  ( -27.00000000000000355, 26.99999999999999645, 12.00000000000000000 ) ) ;
#33587=CARTESIAN_POINT ( 'NONE',  ( 26.99999999999999645, 26.99999999999999645, 0.000000000000000000 ) ) ;
#33617=CARTESIAN_POINT ( 'NONE',  ( -27.00000000000000355, 26.99999999999999289, 15.00000000000000000 ) ) ;
#33803=PLANE ( 'NONE',  #7623 ) ;
#33914=EDGE_CURVE ( 'NONE', #48508, #48281, #50490, .T. ) ;
#34030=DIRECTION ( 'NONE',  ( 0.000000000000000000, 0.000000000000000000, 1.000000000000000000 ) ) ;
#35074=VECTOR ( 'NONE', #3252, 1000.000000000000000 ) ;
#35159=LINE ( 'NONE', #30582, #818 ) ;
#35303=UNCERTAINTY_MEASURE_WITH_UNIT (LENGTH_MEASURE( 1.000000000000000082E-05 ), #55012, 'distance_accuracy_value', 'NONE');
#35598=CARTESIAN_POINT ( 'NONE',  ( -27.00000000000000355, -30.00000000000000355, 0.000000000000000000 ) ) ;
#35711=CIRCLE ( 'NONE', #69382, 2.999999999999999112 ) ;
#35790=ORIENTED_EDGE ( 'NONE', *, *, #19872, .F. ) ;
#36276=AXIS2_PLACEMENT_3D ( 'NONE', #68822, #48739, #4810 ) ;
#36541=ORIENTED_EDGE ( 'NONE', *, *, #63357, .F. ) ;
#36770=VECTOR ( 'NONE', #57032, 1000.000000000000000 ) ;
#36962=CIRCLE ( 'NONE', #65179, 2.999999999999999112 ) ;
#37178=VECTOR ( 'NONE', #16037, 1000.000000000000000 ) ;
#37241=( NAMED_UNIT ( * ) SI_UNIT ( $, .STERADIAN. ) SOLID_ANGLE_UNIT ( ) );
#37456=DIRECTION ( 'NONE',  ( 1.000000000000000000, -0.000000000000000000, -0.000000000000000000 ) ) ;
#37521=ORIENTED_EDGE ( 'NONE', *, *, #63944, .T. ) ;
#37580=CARTESIAN_POINT ( 'NONE',  ( 26.99999999999999645, 26.99999999999999645, 15.00000000000000000 ) ) ;
#37591=SURFACE_STYLE_USAGE ( .BOTH. , #53066 ) ;
#37652=AXIS2_PLACEMENT_3D ( 'NONE', #54094, #658, #43429 ) ;
#37747=PRODUCT ( 'top cover', 'top cover', '', ( #25890 ) ) ;
#37766=FACE_OUTER_BOUND ( 'NONE', #51252, .T. ) ;
#37940=FILL_AREA_STYLE_COLOUR ( '', #55345 ) ;
#37972=DIRECTION ( 'NONE',  ( 0.000000000000000000, 1.000000000000000000, 0.000000000000000000 ) ) ;
#38024=EDGE_CURVE ( 'NONE', #28877, #19323, #64730, .T. ) ;
#38099=CIRCLE ( 'NONE', #66216, 2.999999999999999112 ) ;
#38206=FACE_BOUND ( 'NONE', #63415, .T. ) ;
#38318=ORIENTED_EDGE ( 'NONE', *, *, #2303, .T. ) ;
#38738=VECTOR ( 'NONE', #50391, 1000.000000000000000 ) ;
#38878=ORIENTED_EDGE ( 'NONE', *, *, #4241, .F. ) ;
#38884=PLANE ( 'NONE',  #5366 ) ;
#38910=DIRECTION ( 'NONE',  ( -1.000000000000000000, 0.000000000000000000, 0.000000000000000000 ) ) ;
#39077=DIRECTION ( 'NONE',  ( -1.000000000000000000, 0.000000000000000000, -0.000000000000000000 ) ) ;
#39225=ORIENTED_EDGE ( 'NONE', *, *, #18804, .T. ) ;
#39230=ORIENTED_EDGE ( 'NONE', *, *, #12281, .F. ) ;
#39545=( NAMED_UNIT ( * ) PLANE_ANGLE_UNIT ( ) SI_UNIT ( $, .RADIAN. ) );
#39573=VERTEX_POINT ( 'NONE', #59829 ) ;
#39605=CARTESIAN_POINT ( 'NONE',  ( -27.00000000000000355, 26.99999999999999645, 12.00000000000000000 ) ) ;
#39638=ORIENTED_EDGE ( 'NONE', *, *, #41836, .F. ) ;
#39648=CARTESIAN_POINT ( 'NONE',  ( 26.99999999999999645, 26.99999999999999645, 12.00000000000000000 ) ) ;
#39825=ORIENTED_EDGE ( 'NONE', *, *, #66739, .F. ) ;
#39830=SPHERICAL_SURFACE ( 'NONE', #26860, 3.000000000000000000 ) ;
#39889=AXIS2_PLACEMENT_3D ( 'NONE', #18189, #40671, #29777 ) ;
#40175=VERTEX_POINT ( 'NONE', #232 ) ;
#40671=DIRECTION ( 'NONE',  ( 0.000000000000000000, -1.000000000000000000, 0.000000000000000000 ) ) ;
#40685=CARTESIAN_POINT ( 'NONE',  ( -27.00000000000000355, -27.00000000000000355, 12.00000000000000000 ) ) ;
#40909=VECTOR ( 'NONE', #32096, 1000.000000000000000 ) ;
#41051=ORIENTED_EDGE ( 'NONE', *, *, #21428, .T. ) ;
#41140=CARTESIAN_POINT ( 'NONE',  ( 26.99999999999999645, -27.00000000000000355, 12.00000000000000000 ) ) ;
#41231=VECTOR ( 'NONE', #60463, 1000.000000000000000 ) ;
#41324=VERTEX_POINT ( 'NONE', #33587 ) ;
#41397=FACE_OUTER_BOUND ( 'NONE', #56560, .T. ) ;
#41457=EDGE_CURVE ( 'NONE', #43408, #7667, #20503, .T. ) ;
#41498=FACE_OUTER_BOUND ( 'NONE', #43174, .T. ) ;
#41537=LINE ( 'NONE', #57715, #13179 ) ;
#41647=CARTESIAN_POINT ( 'NONE',  ( -27.00000000000000355, 26.99999999999999645, 15.00000000000000000 ) ) ;
#41781=FACE_OUTER_BOUND ( 'NONE', #68057, .T. ) ;
#41836=EDGE_CURVE ( 'NONE', #32499, #9081, #13919, .T. ) ;
#41986=DIRECTION ( 'NONE',  ( 0.000000000000000000, 0.000000000000000000, -1.000000000000000000 ) ) ;
#42212=EDGE_LOOP ( 'NONE', ( #26423, #52537, #65049, #60147 ) ) ;
#42318=VERTEX_POINT ( 'NONE', #37580 ) ;
#42447=PLANE ( 'NONE',  #14925 ) ;
#42477=EDGE_CURVE ( 'NONE', #42318, #32375, #24075, .T. ) ;
#42563=LINE ( 'NONE', #31331, #58896 ) ;
#42592=ORIENTED_EDGE ( 'NONE', *, *, #9480, .F. ) ;
#42715=ORIENTED_EDGE ( 'NONE', *, *, #42477, .F. ) ;
#42893=CLOSED_SHELL ( 'NONE', ( #21321, #26910, #50343, #65857, #27010, #8423, #12964, #28319, #61135, #21352, #53679, #9857, #10700, #21422, #24695, #13635, #32965, #3439, #45010, #10784, #31914, #20784, #12906 ) ) ;
#42919=VECTOR ( 'NONE', #16540, 1000.000000000000000 ) ;
#43010=ORIENTED_EDGE ( 'NONE', *, *, #65275, .T. ) ;
#43158=EDGE_LOOP ( 'NONE', ( #56517, #21082, #14630 ) ) ;
#43174=EDGE_LOOP ( 'NONE', ( #46966, #50218, #54926, #5803 ) ) ;
#43201=( NAMED_UNIT ( * ) PLANE_ANGLE_UNIT ( ) SI_UNIT ( $, .RADIAN. ) );
#43408=VERTEX_POINT ( 'NONE', #30781 ) ;
#43429=DIRECTION ( 'NONE',  ( 0.000000000000000000, -0.000000000000000000, 1.000000000000000000 ) ) ;
#43473=CYLINDRICAL_SURFACE ( 'NONE', #36276, 2.999999999999999112 ) ;
#43721=CARTESIAN_POINT ( 'NONE',  ( 29.99999999999999645, -27.00000000000000355, 12.00000000000000000 ) ) ;
#43751=EDGE_CURVE ( 'NONE', #69327, #32375, #15172, .T. ) ;
#43898=AXIS2_PLACEMENT_3D ( 'NONE', #39605, #55072, #22375 ) ;
#43899=PLANE ( 'NONE',  #53069 ) ;
#44096=CARTESIAN_POINT ( 'NONE',  ( 26.99999999999999289, -30.00000000000000355, 15.00000000000000000 ) ) ;
#44273=EDGE_LOOP ( 'NONE', ( #46666, #11039, #2102, #710 ) ) ;
#44558=DIRECTION ( 'NONE',  ( 0.000000000000000000, 0.000000000000000000, 1.000000000000000000 ) ) ;
#44685=LINE ( 'NONE', #16893, #27182 ) ;
#44764=EDGE_LOOP ( 'NONE', ( #59766, #13708, #3891, #50108 ) ) ;
#44835=DIRECTION ( 'NONE',  ( -0.000000000000000000, 0.000000000000000000, 1.000000000000000000 ) ) ;
#44857=CARTESIAN_POINT ( 'NONE',  ( 29.99999999999999645, 26.99999999999999289, 0.000000000000000000 ) ) ;
#44883=DIRECTION ( 'NONE',  ( 0.000000000000000000, 0.000000000000000000, -1.000000000000000000 ) ) ;
#44889=VERTEX_POINT ( 'NONE', #43721 ) ;
#45010=ADVANCED_FACE ( 'NONE', ( #37766 ), #27909, .T. ) ;
#45161=DIRECTION ( 'NONE',  ( 0.000000000000000000, 1.000000000000000000, 0.000000000000000000 ) ) ;
#45182=LINE ( 'NONE', #19485, #14733 ) ;
#45225=DIRECTION ( 'NONE',  ( -0.000000000000000000, 1.000000000000000000, -0.000000000000000000 ) ) ;
#45423=LINE ( 'NONE', #8141, #29640 ) ;
#45523=DIRECTION ( 'NONE',  ( 1.000000000000000000, 0.000000000000000000, 0.000000000000000000 ) ) ;
#45780=CARTESIAN_POINT ( 'NONE',  ( -30.00000000000000355, 26.99999999999999289, 15.00000000000000000 ) ) ;
#46098=AXIS2_PLACEMENT_3D ( 'NONE', #56522, #51263, #4446 ) ;
#46224=DIRECTION ( 'NONE',  ( 1.000000000000000000, 0.000000000000000000, 0.000000000000000000 ) ) ;
#46448=CARTESIAN_POINT ( 'NONE',  ( 26.99999999999999645, -27.00000000000000355, 0.000000000000000000 ) ) ;
#46485=EDGE_LOOP ( 'NONE', ( #51550, #29677, #64512, #35790 ) ) ;
#46666=ORIENTED_EDGE ( 'NONE', *, *, #41457, .T. ) ;
#46788=EDGE_CURVE ( 'NONE', #42318, #6225, #11217, .T. ) ;
#46794=EDGE_CURVE ( 'NONE', #32375, #51688, #60101, .T. ) ;
#46841=EDGE_CURVE ( 'NONE', #44889, #51452, #10889, .T. ) ;
#46966=ORIENTED_EDGE ( 'NONE', *, *, #43751, .F. ) ;
#47075=CARTESIAN_POINT ( 'NONE',  ( -30.00000000000000355, 26.99999999999999289, 0.000000000000000000 ) ) ;
#47081=FACE_OUTER_BOUND ( 'NONE', #16158, .T. ) ;
#47199=LINE ( 'NONE', #14846, #13692 ) ;
#47440=DIRECTION ( 'NONE',  ( 0.000000000000000000, 0.000000000000000000, -1.000000000000000000 ) ) ;
#47705=AXIS2_PLACEMENT_3D ( 'NONE', #26000, #31962, #53389 ) ;
#47729=DIRECTION ( 'NONE',  ( 1.000000000000000000, -0.000000000000000000, 0.000000000000000000 ) ) ;
#47841=AXIS2_PLACEMENT_3D ( 'NONE', #11030, #26528, #64853 ) ;
#47934=ORIENTED_EDGE ( 'NONE', *, *, #2303, .F. ) ;
#47952=AXIS2_PLACEMENT_3D ( 'NONE', #22018, #205, #49429 ) ;
#48125=LINE ( 'NONE', #62944, #29954 ) ;
#48281=VERTEX_POINT ( 'NONE', #21793 ) ;
#48385=CARTESIAN_POINT ( 'NONE',  ( 26.99999999999999645, -27.00000000000000355, 12.00000000000000000 ) ) ;
#48462=( LENGTH_UNIT ( ) NAMED_UNIT ( * ) SI_UNIT ( .MILLI., .METRE. ) );
#48508=VERTEX_POINT ( 'NONE', #47075 ) ;
#48624=VECTOR ( 'NONE', #31081, 1000.000000000000000 ) ;
#48692=VECTOR ( 'NONE', #37456, 1000.000000000000000 ) ;
#48704=DIRECTION ( 'NONE',  ( 0.000000000000000000, 0.000000000000000000, -1.000000000000000000 ) ) ;
#48739=DIRECTION ( 'NONE',  ( -1.000000000000000000, 0.000000000000000000, 0.000000000000000000 ) ) ;
#48816=FACE_OUTER_BOUND ( 'NONE', #44273, .T. ) ;
#48833=DIRECTION ( 'NONE',  ( -1.000000000000000000, 0.000000000000000000, 0.000000000000000000 ) ) ;
#48857=DIRECTION ( 'NONE',  ( -1.000000000000000000, 0.000000000000000000, 0.000000000000000000 ) ) ;
#49116=DIRECTION ( 'NONE',  ( 1.000000000000000000, 0.000000000000000000, 0.000000000000000000 ) ) ;
#49201=CARTESIAN_POINT ( 'NONE',  ( -27.00000000000000355, -27.00000000000000355, 12.00000000000000000 ) ) ;
#49429=DIRECTION ( 'NONE',  ( -1.000000000000000000, 0.000000000000000000, 0.000000000000000000 ) ) ;
#49518=ORIENTED_EDGE ( 'NONE', *, *, #33914, .F. ) ;
#49892=CARTESIAN_POINT ( 'NONE',  ( 0.000000000000000000, 0.000000000000000000, 15.00000000000000000 ) ) ;
#49910=DIRECTION ( 'NONE',  ( 0.000000000000000000, -1.000000000000000000, 0.000000000000000000 ) ) ;
#49967=AXIS2_PLACEMENT_3D ( 'NONE', #22720, #38910, #54718 ) ;
#50099=( NAMED_UNIT ( * ) SI_UNIT ( $, .STERADIAN. ) SOLID_ANGLE_UNIT ( ) );
#50108=ORIENTED_EDGE ( 'NONE', *, *, #3314, .F. ) ;
#50132=AXIS2_PLACEMENT_3D ( 'NONE', #32203, #6143, #21294 ) ;
#50218=ORIENTED_EDGE ( 'NONE', *, *, #62047, .F. ) ;
#50333=DIRECTION ( 'NONE',  ( 0.000000000000000000, -1.000000000000000000, 0.000000000000000000 ) ) ;
#50343=ADVANCED_FACE ( 'NONE', ( #18121 ), #38884, .F. ) ;
#50391=DIRECTION ( 'NONE',  ( -0.000000000000000000, -0.000000000000000000, 1.000000000000000000 ) ) ;
#50443=EDGE_CURVE ( 'NONE', #7667, #64962, #35711, .T. ) ;
#50490=CIRCLE ( 'NONE', #58354, 2.999999999999999112 ) ;
#50530=CARTESIAN_POINT ( 'NONE',  ( 0.000000000000000000, 0.000000000000000000, 0.000000000000000000 ) ) ;
#50672=DIRECTION ( 'NONE',  ( 1.000000000000000000, -0.000000000000000000, 0.000000000000000000 ) ) ;
#50724=EDGE_CURVE ( 'NONE', #48508, #8633, #8001, .T. ) ;
#50736=EDGE_CURVE ( 'NONE', #58514, #25791, #25918, .T. ) ;
#50808=DIRECTION ( 'NONE',  ( -0.000000000000000000, -0.000000000000000000, 1.000000000000000000 ) ) ;
#51010=ORIENTED_EDGE ( 'NONE', *, *, #64649, .F. ) ;
#51145=DIRECTION ( 'NONE',  ( 0.000000000000000000, 0.000000000000000000, 1.000000000000000000 ) ) ;
#51252=EDGE_LOOP ( 'NONE', ( #53314, #6889, #1414, #42592 ) ) ;
#51256=ORIENTED_EDGE ( 'NONE', *, *, #25060, .T. ) ;
#51263=DIRECTION ( 'NONE',  ( 1.000000000000000000, 0.000000000000000000, 0.000000000000000000 ) ) ;
#51452=VERTEX_POINT ( 'NONE', #58770 ) ;
#51494=VECTOR ( 'NONE', #21320, 1000.000000000000000 ) ;
#51550=ORIENTED_EDGE ( 'NONE', *, *, #6516, .T. ) ;
#51688=VERTEX_POINT ( 'NONE', #26357 ) ;
#52083=EDGE_CURVE ( 'NONE', #41324, #6058, #47199, .T. ) ;
#52460=VERTEX_POINT ( 'NONE', #58699 ) ;
#52496=ORIENTED_EDGE ( 'NONE', *, *, #62047, .T. ) ;
#52537=ORIENTED_EDGE ( 'NONE', *, *, #18804, .F. ) ;
#52604=LINE ( 'NONE', #27248, #48692 ) ;
#52619=AXIS2_PLACEMENT_3D ( 'NONE', #20346, #26668, #26328 ) ;
#52751=ORIENTED_EDGE ( 'NONE', *, *, #46841, .T. ) ;
#52946=EDGE_LOOP ( 'NONE', ( #56917, #52751, #39825 ) ) ;
#53066=SURFACE_SIDE_STYLE ('',( #27377 ) ) ;
#53069=AXIS2_PLACEMENT_3D ( 'NONE', #53756, #298, #31631 ) ;
#53074=AXIS2_PLACEMENT_3D ( 'NONE', #19469, #45161, #51145 ) ;
#53306=CARTESIAN_POINT ( 'NONE',  ( 26.99999999999999645, 0.000000000000000000, 12.00000000000000000 ) ) ;
#53314=ORIENTED_EDGE ( 'NONE', *, *, #63944, .F. ) ;
#53339=ORIENTED_EDGE ( 'NONE', *, *, #24976, .F. ) ;
#53389=DIRECTION ( 'NONE',  ( 0.000000000000000000, 1.156482317317871725E-15, 1.000000000000000000 ) ) ;
#53679=ADVANCED_FACE ( 'NONE', ( #2271 ), #8234, .T. ) ;
#53756=CARTESIAN_POINT ( 'NONE',  ( -30.00000000000000355, -27.00000000000000355, 15.00000000000000000 ) ) ;
#53849=ORIENTED_EDGE ( 'NONE', *, *, #32658, .F. ) ;
#53871=CARTESIAN_POINT ( 'NONE',  ( 29.99999999999999645, -30.00000000000000355, 12.00000000000000000 ) ) ;
#54094=CARTESIAN_POINT ( 'NONE',  ( -30.00000000000000355, -30.00000000000000355, 15.00000000000000000 ) ) ;
#54138=CARTESIAN_POINT ( 'NONE',  ( 26.99999999999999645, -27.00000000000000355, 0.000000000000000000 ) ) ;
#54277=EDGE_LOOP ( 'NONE', ( #33220, #56081, #19413, #60584 ) ) ;
#54510=EDGE_CURVE ( 'NONE', #52460, #32375, #52604, .T. ) ;
#54516=DIRECTION ( 'NONE',  ( 0.000000000000000000, 0.000000000000000000, -1.000000000000000000 ) ) ;
#54598=DIRECTION ( 'NONE',  ( -0.000000000000000000, 1.000000000000000000, 0.000000000000000000 ) ) ;
#54718=DIRECTION ( 'NONE',  ( 0.000000000000000000, 0.000000000000000000, 1.000000000000000000 ) ) ;
#54767=DIRECTION ( 'NONE',  ( -0.000000000000000000, -1.000000000000000000, -0.000000000000000000 ) ) ;
#54871=ORIENTED_EDGE ( 'NONE', *, *, #66115, .F. ) ;
#54926=ORIENTED_EDGE ( 'NONE', *, *, #65993, .F. ) ;
#55012=( LENGTH_UNIT ( ) NAMED_UNIT ( * ) SI_UNIT ( .MILLI., .METRE. ) );
#55072=DIRECTION ( 'NONE',  ( -1.000000000000000000, 0.000000000000000000, 0.000000000000000000 ) ) ;
#55165=DIRECTION ( 'NONE',  ( 0.000000000000000000, 0.000000000000000000, -1.000000000000000000 ) ) ;
#55232=DIRECTION ( 'NONE',  ( 0.000000000000000000, 0.000000000000000000, -1.000000000000000000 ) ) ;
#55345=COLOUR_RGB ( '',0.7921568627450980005, 0.8196078431372548767, 0.9333333333333333481 ) ;
#55427=DIRECTION ( 'NONE',  ( -0.000000000000000000, 1.000000000000000000, 0.000000000000000000 ) ) ;
#55459=CIRCLE ( 'NONE', #25151, 2.999999999999999112 ) ;
#55565=PRODUCT_DEFINITION ( 'UNKNOWN', '', #32152, #9955 ) ;
#55660=FACE_OUTER_BOUND ( 'NONE', #3101, .T. ) ;
#55869=VERTEX_POINT ( 'NONE', #33528 ) ;
#55920=EDGE_CURVE ( 'NONE', #48281, #52460, #65890, .T. ) ;
#56081=ORIENTED_EDGE ( 'NONE', *, *, #9480, .T. ) ;
#56192=EDGE_LOOP ( 'NONE', ( #39638, #53849, #53339, #39230 ) ) ;
#56517=ORIENTED_EDGE ( 'NONE', *, *, #16118, .T. ) ;
#56522=CARTESIAN_POINT ( 'NONE',  ( -30.00000000000000355, -30.00000000000000355, 15.00000000000000000 ) ) ;
#56560=EDGE_LOOP ( 'NONE', ( #14415, #39225, #41051, #27068 ) ) ;
#56589=ORIENTED_EDGE ( 'NONE', *, *, #30023, .F. ) ;
#56624=DIRECTION ( 'NONE',  ( -1.000000000000000000, -0.000000000000000000, 0.000000000000000000 ) ) ;
#56670=CARTESIAN_POINT ( 'NONE',  ( -27.00000000000000355, -27.00000000000000355, 0.000000000000000000 ) ) ;
#56917=ORIENTED_EDGE ( 'NONE', *, *, #24976, .T. ) ;
#57032=DIRECTION ( 'NONE',  ( 0.000000000000000000, 0.000000000000000000, -1.000000000000000000 ) ) ;
#57340=DIRECTION ( 'NONE',  ( 0.000000000000000000, 1.000000000000000000, 0.000000000000000000 ) ) ;
#57397=LINE ( 'NONE', #18380, #35074 ) ;
#57437=CIRCLE ( 'NONE', #43898, 2.999999999999999112 ) ;
#57491=ORIENTED_EDGE ( 'NONE', *, *, #33914, .T. ) ;
#57715=CARTESIAN_POINT ( 'NONE',  ( 0.000000000000000000, -27.00000000000000355, 12.00000000000000000 ) ) ;
#57909=PLANE ( 'NONE',  #46098 ) ;
#58354=AXIS2_PLACEMENT_3D ( 'NONE', #5648, #5318, #31705 ) ;
#58355=PRESENTATION_STYLE_ASSIGNMENT (( #37591 ) ) ;
#58514=VERTEX_POINT ( 'NONE', #31628 ) ;
#58699=CARTESIAN_POINT ( 'NONE',  ( -27.00000000000000355, 29.99999999999999645, 12.00000000000000000 ) ) ;
#58756=EDGE_CURVE ( 'NONE', #7667, #39573, #7471, .T. ) ;
#58769=APPLICATION_CONTEXT ( 'automotive_design' ) ;
#58770=CARTESIAN_POINT ( 'NONE',  ( 26.99999999999999645, -27.00000000000000355, 15.00000000000000000 ) ) ;
#58799=VECTOR ( 'NONE', #63234, 1000.000000000000000 ) ;
#58842=LINE ( 'NONE', #5040, #62828 ) ;
#58896=VECTOR ( 'NONE', #25714, 1000.000000000000000 ) ;
#59013=ORIENTED_EDGE ( 'NONE', *, *, #50736, .F. ) ;
#59647=FACE_OUTER_BOUND ( 'NONE', #28482, .T. ) ;
#59754=VERTEX_POINT ( 'NONE', #46448 ) ;
#59766=ORIENTED_EDGE ( 'NONE', *, *, #64649, .T. ) ;
#59829=CARTESIAN_POINT ( 'NONE',  ( -27.00000000000000355, -27.00000000000000355, 15.00000000000000000 ) ) ;
#60101=LINE ( 'NONE', #28096, #41231 ) ;
#60147=ORIENTED_EDGE ( 'NONE', *, *, #23029, .F. ) ;
#60293=LINE ( 'NONE', #6823, #5733 ) ;
#60299=ORIENTED_EDGE ( 'NONE', *, *, #19872, .T. ) ;
#60331=LINE ( 'NONE', #33617, #11234 ) ;
#60441=ORIENTED_EDGE ( 'NONE', *, *, #23205, .F. ) ;
#60463=DIRECTION ( 'NONE',  ( 0.000000000000000000, 0.000000000000000000, -1.000000000000000000 ) ) ;
#60584=ORIENTED_EDGE ( 'NONE', *, *, #66115, .T. ) ;
#60813=DIRECTION ( 'NONE',  ( 0.000000000000000000, 0.000000000000000000, -1.000000000000000000 ) ) ;
#60843=DIRECTION ( 'NONE',  ( -1.000000000000000000, 0.000000000000000000, 0.000000000000000000 ) ) ;
#60872=DIRECTION ( 'NONE',  ( 0.000000000000000000, -0.000000000000000000, -1.000000000000000000 ) ) ;
#60935=CARTESIAN_POINT ( 'NONE',  ( -27.00000000000000355, 29.99999999999999645, 15.00000000000000000 ) ) ;
#60954=ORIENTED_EDGE ( 'NONE', *, *, #41836, .T. ) ;
#61026=LINE ( 'NONE', #13198, #19906 ) ;
#61135=ADVANCED_FACE ( 'NONE', ( #65243 ), #26232, .T. ) ;
#61229=FACE_OUTER_BOUND ( 'NONE', #13156, .T. ) ;
#61971=ORIENTED_EDGE ( 'NONE', *, *, #17309, .F. ) ;
#62047=EDGE_CURVE ( 'NONE', #62713, #69327, #61026, .T. ) ;
#62100=ORIENTED_EDGE ( 'NONE', *, *, #30420, .F. ) ;
#62196=VECTOR ( 'NONE', #1463, 1000.000000000000000 ) ;
#62265=CYLINDRICAL_SURFACE ( 'NONE', #25812, 2.999999999999999112 ) ;
#62336=EDGE_CURVE ( 'NONE', #26503, #9081, #35159, .T. ) ;
#62459=ORIENTED_EDGE ( 'NONE', *, *, #54510, .F. ) ;
#62596=VECTOR ( 'NONE', #6825, 1000.000000000000000 ) ;
#62713=VERTEX_POINT ( 'NONE', #44857 ) ;
#62828=VECTOR ( 'NONE', #41986, 1000.000000000000000 ) ;
#62893=SPHERICAL_SURFACE ( 'NONE', #17522, 3.000000000000000000 ) ;
#62900=CARTESIAN_POINT ( 'NONE',  ( 29.99999999999999645, 26.99999999999999645, 12.00000000000000000 ) ) ;
#62944=CARTESIAN_POINT ( 'NONE',  ( 26.99999999999999645, 26.99999999999999289, 15.00000000000000000 ) ) ;
#62949=CARTESIAN_POINT ( 'NONE',  ( 26.99999999999999289, 26.99999999999999645, 15.00000000000000000 ) ) ;
#62997=VECTOR ( 'NONE', #25582, 1000.000000000000000 ) ;
#63234=DIRECTION ( 'NONE',  ( 1.000000000000000000, 0.000000000000000000, 0.000000000000000000 ) ) ;
#63307=ORIENTED_EDGE ( 'NONE', *, *, #52083, .T. ) ;
#63343=DIRECTION ( 'NONE',  ( 0.000000000000000000, 1.000000000000000000, 0.000000000000000000 ) ) ;
#63357=EDGE_CURVE ( 'NONE', #51688, #48281, #14417, .T. ) ;
#63415=EDGE_LOOP ( 'NONE', ( #38318, #5156, #37521, #63307 ) ) ;
#63944=EDGE_CURVE ( 'NONE', #59754, #41324, #25689, .T. ) ;
#63984=FACE_OUTER_BOUND ( 'NONE', #27696, .T. ) ;
#64245=CIRCLE ( 'NONE', #27026, 2.999999999999999112 ) ;
#64363=CARTESIAN_POINT ( 'NONE',  ( 29.99999999999999645, -30.00000000000000355, 0.000000000000000000 ) ) ;
#64512=ORIENTED_EDGE ( 'NONE', *, *, #33002, .F. ) ;
#64643=AXIS2_PLACEMENT_3D ( 'NONE', #28660, #44835, #45523 ) ;
#64649=EDGE_CURVE ( 'NONE', #69327, #42318, #14478, .T. ) ;
#64730=LINE ( 'NONE', #22511, #42919 ) ;
#64825=EDGE_LOOP ( 'NONE', ( #7438, #59013, #4008, #43010 ) ) ;
#64853=DIRECTION ( 'NONE',  ( 0.000000000000000000, 0.000000000000000000, 1.000000000000000000 ) ) ;
#64962=VERTEX_POINT ( 'NONE', #12484 ) ;
#65049=ORIENTED_EDGE ( 'NONE', *, *, #4904, .F. ) ;
#65063=AXIS2_PLACEMENT_3D ( 'NONE', #62949, #47440, #14758 ) ;
#65179=AXIS2_PLACEMENT_3D ( 'NONE', #15349, #48704, #20967 ) ;
#65243=FACE_OUTER_BOUND ( 'NONE', #27456, .T. ) ;
#65275=EDGE_CURVE ( 'NONE', #19323, #55869, #1860, .T. ) ;
#65623=AXIS2_PLACEMENT_3D ( 'NONE', #1835, #22231, #28196 ) ;
#65637=CYLINDRICAL_SURFACE ( 'NONE', #47952, 2.999999999999999112 ) ;
#65745=AXIS2_PLACEMENT_3D ( 'NONE', #10261, #24734, #67992 ) ;
#65857=ADVANCED_FACE ( 'NONE', ( #41397 ), #57909, .F. ) ;
#65890=LINE ( 'NONE', #60935, #38738 ) ;
#65979=CARTESIAN_POINT ( 'NONE',  ( -30.00000000000000355, 29.99999999999999645, 15.00000000000000000 ) ) ;
#65993=EDGE_CURVE ( 'NONE', #51688, #62713, #36962, .T. ) ;
#66068=ORIENTED_EDGE ( 'NONE', *, *, #4904, .T. ) ;
#66101=FACE_OUTER_BOUND ( 'NONE', #15255, .T. ) ;
#66114=DIRECTION ( 'NONE',  ( 0.000000000000000000, -1.000000000000000000, 0.000000000000000000 ) ) ;
#66115=EDGE_CURVE ( 'NONE', #55869, #6058, #60331, .T. ) ;
#66185=DIRECTION ( 'NONE',  ( 0.000000000000000000, 0.000000000000000000, 1.000000000000000000 ) ) ;
#66216=AXIS2_PLACEMENT_3D ( 'NONE', #17561, #49910, #60813 ) ;
#66427=DIRECTION ( 'NONE',  ( -1.156482317317871725E-15, 0.000000000000000000, -1.000000000000000000 ) ) ;
#66522=DIRECTION ( 'NONE',  ( -1.000000000000000000, 0.000000000000000000, 0.000000000000000000 ) ) ;
#66647=EDGE_CURVE ( 'NONE', #58514, #59754, #44685, .T. ) ;
#66655=DIRECTION ( 'NONE',  ( 0.000000000000000000, 1.000000000000000000, 0.000000000000000000 ) ) ;
#66739=EDGE_CURVE ( 'NONE', #43408, #51452, #64245, .T. ) ;
#66771=DIRECTION ( 'NONE',  ( -1.000000000000000000, -0.000000000000000000, 1.156482317317871725E-15 ) ) ;
#66832=AXIS2_PLACEMENT_3D ( 'NONE', #50530, #44558, #8319 ) ;
#67585=DIRECTION ( 'NONE',  ( 1.000000000000000000, -0.000000000000000000, 0.000000000000000000 ) ) ;
#67719=MECHANICAL_DESIGN_GEOMETRIC_PRESENTATION_REPRESENTATION('',(#24993),#16028);
#67958=ORIENTED_EDGE ( 'NONE', *, *, #66739, .T. ) ;
#67992=DIRECTION ( 'NONE',  ( 1.000000000000000000, 0.000000000000000000, 0.000000000000000000 ) ) ;
#68057=EDGE_LOOP ( 'NONE', ( #51010, #26389, #42715 ) ) ;
#68427=ORIENTED_EDGE ( 'NONE', *, *, #41457, .F. ) ;
#68449=SHAPE_DEFINITION_REPRESENTATION ( #9074, #31639 ) ;
#68822=CARTESIAN_POINT ( 'NONE',  ( 0.000000000000000000, 26.99999999999999645, 12.00000000000000000 ) ) ;
#68838=DIRECTION ( 'NONE',  ( 0.000000000000000000, 0.000000000000000000, 1.000000000000000000 ) ) ;
#69310=ORIENTED_EDGE ( 'NONE', *, *, #32658, .T. ) ;
#69315=DIRECTION ( 'NONE',  ( 0.000000000000000000, 0.000000000000000000, -1.000000000000000000 ) ) ;
#69327=VERTEX_POINT ( 'NONE', #62900 ) ;
#69382=AXIS2_PLACEMENT_3D ( 'NONE', #30400, #3324, #46224 ) ;
ENDSEC;
END-ISO-10303-21;
